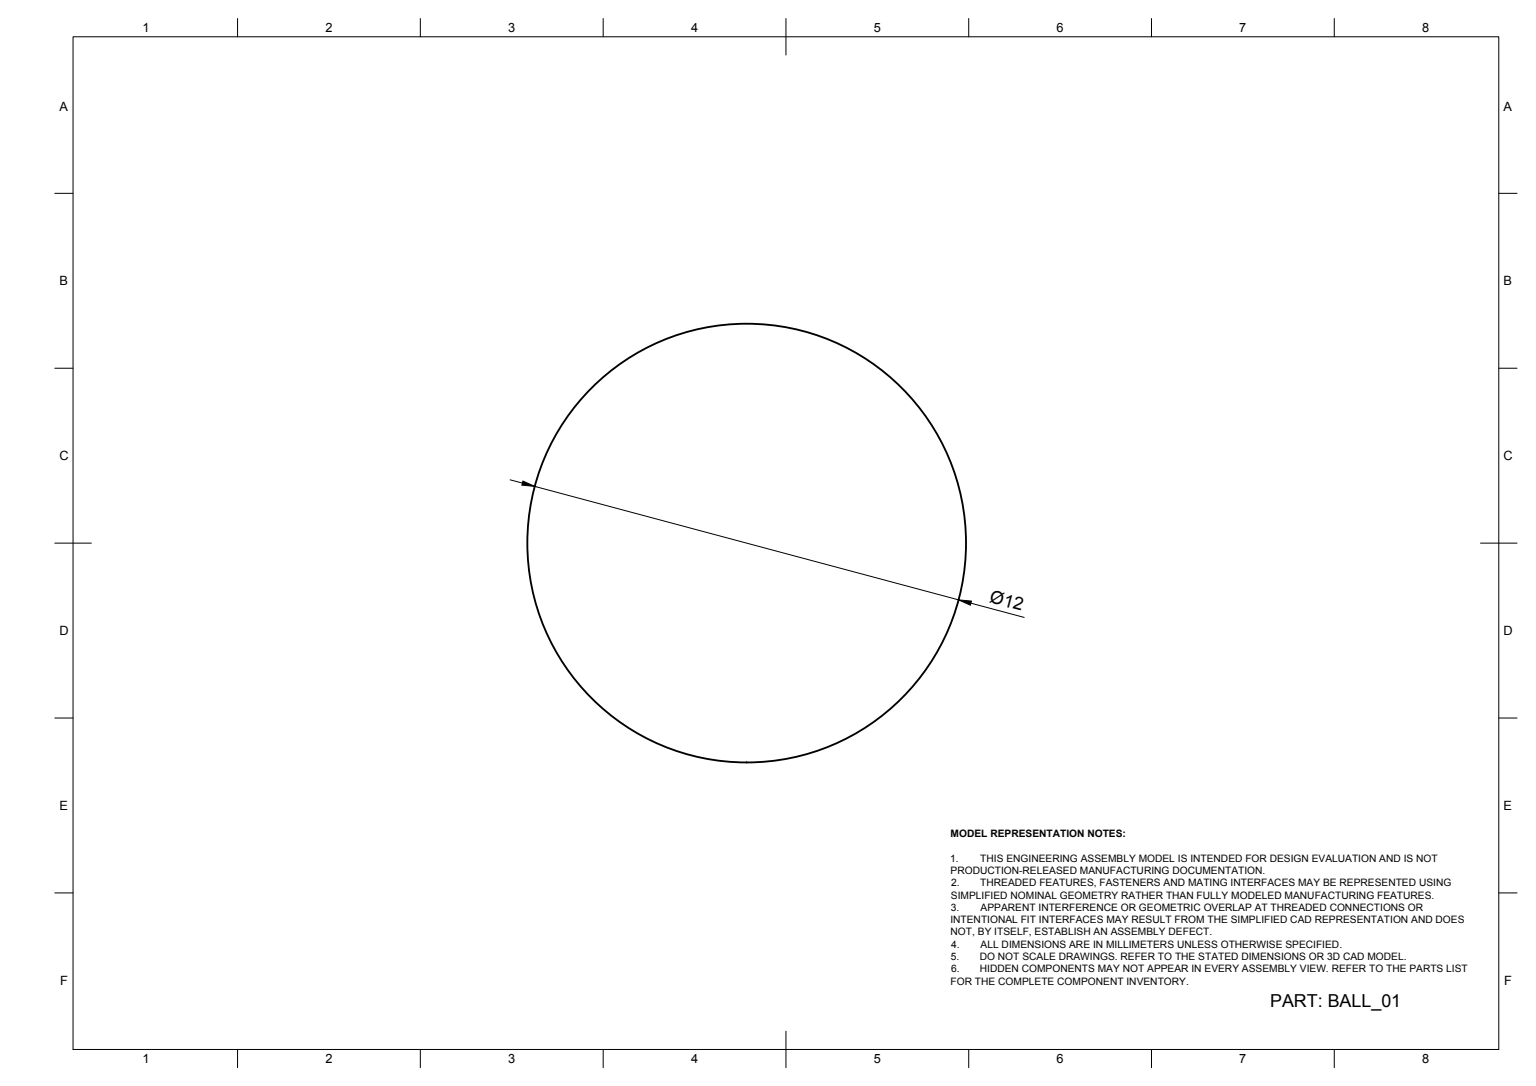
ISO-10303-21;
HEADER;
/* Generated by software containing ST-Developer
 * from STEP Tools, Inc. (www.steptools.com) 
 */

FILE_DESCRIPTION(
/* description */ (''),
/* implementation_level */ '2;1');

FILE_NAME(
/* name */ 'Ball_01.step',
/* time_stamp */ '2026-10-05T00:14:20-07:00',
/* author */ (''),
/* organization */ (''),
/* preprocessor_version */ 'ST-DEVELOPER v20.2',
/* originating_system */ 'Autodesk Translation Framework v15.15.0.0',
/* authorisation */ '');

FILE_SCHEMA (('AUTOMOTIVE_DESIGN { 1 0 10303 214 3 1 1 }'));
ENDSEC;

DATA;
#10=MECHANICAL_DESIGN_GEOMETRIC_PRESENTATION_REPRESENTATION('',(#3372),#75336);
#3352=SPHERICAL_SURFACE('',#32135,6.);
#3356=SHAPE_REPRESENTATION_RELATIONSHIP('SRR','None',#75369,#3364);
#3364=ADVANCED_BREP_SHAPE_REPRESENTATION('',(#3380),#75329);
#3372=STYLED_ITEM('',(#75418),#3380);
#3380=MANIFOLD_SOLID_BREP('Body1',#32022);
#3402=CIRCLE('',#32136,6.);
#5146=FACE_OUTER_BOUND('',#6874,.T.);
#6874=EDGE_LOOP('',(#19625,#19626));
#11108=VERTEX_POINT('',#46100);
#11109=VERTEX_POINT('',#46101);
#14507=EDGE_CURVE('',#11108,#11109,#3402,.T.);
#19625=ORIENTED_EDGE('',*,*,#14507,.T.);
#19626=ORIENTED_EDGE('',*,*,#14507,.F.);
#30306=ADVANCED_FACE('',(#5146),#3352,.T.);
#32022=CLOSED_SHELL('',(#30306));
#32134=AXIS2_PLACEMENT_3D('',#46098,#36399,#36400);
#32135=AXIS2_PLACEMENT_3D('',#46099,#36401,#36402);
#32136=AXIS2_PLACEMENT_3D('',#46102,#36403,#36404);
#36399=DIRECTION('axis',(0.,0.,1.));
#36400=DIRECTION('refdir',(1.,0.,0.));
#36401=DIRECTION('center_axis',(0.,0.,1.));
#36402=DIRECTION('ref_axis',(1.,0.,0.));
#36403=DIRECTION('center_axis',(1.22464679914735E-16,-1.,0.));
#36404=DIRECTION('ref_axis',(-1.,-1.22464679914735E-16,0.));
#46098=CARTESIAN_POINT('',(0.,0.,0.));
#46099=CARTESIAN_POINT('Origin',(30.,-9.99200722162641E-15,13.));
#46100=CARTESIAN_POINT('',(30.,-9.99200722162641E-15,19.));
#46101=CARTESIAN_POINT('',(30.,-9.99200722162641E-15,7.));
#46102=CARTESIAN_POINT('Origin',(30.,-9.99200722162641E-15,13.));
#75319=UNCERTAINTY_MEASURE_WITH_UNIT(LENGTH_MEASURE(0.01),#75337,
'DISTANCE_ACCURACY_VALUE',
'Maximum model space distance between geometric entities at asserted c
onnectivities');
#75326=UNCERTAINTY_MEASURE_WITH_UNIT(LENGTH_MEASURE(0.01),#75337,
'DISTANCE_ACCURACY_VALUE',
'Maximum model space distance between geometric entities at asserted c
onnectivities');
#75329=(
GEOMETRIC_REPRESENTATION_CONTEXT(3)
GLOBAL_UNCERTAINTY_ASSIGNED_CONTEXT((#75319))
GLOBAL_UNIT_ASSIGNED_CONTEXT((#75337,#75339,#75340))
REPRESENTATION_CONTEXT('','3D')
);
#75336=(
GEOMETRIC_REPRESENTATION_CONTEXT(3)
GLOBAL_UNCERTAINTY_ASSIGNED_CONTEXT((#75326))
GLOBAL_UNIT_ASSIGNED_CONTEXT((#75337,#75339,#75340))
REPRESENTATION_CONTEXT('','3D')
);
#75337=(
LENGTH_UNIT()
NAMED_UNIT(*)
SI_UNIT(.MILLI.,.METRE.)
);
#75339=(
NAMED_UNIT(*)
PLANE_ANGLE_UNIT()
SI_UNIT($,.RADIAN.)
);
#75340=(
NAMED_UNIT(*)
SI_UNIT($,.STERADIAN.)
SOLID_ANGLE_UNIT()
);
#75343=SHAPE_DEFINITION_REPRESENTATION(#75352,#75369);
#75352=PRODUCT_DEFINITION_SHAPE('',$,#75379);
#75369=SHAPE_REPRESENTATION('',(#32134),#75329);
#75376=PRODUCT_DEFINITION_CONTEXT('part definition',#75405,'design');
#75379=PRODUCT_DEFINITION('Ball_01','Ball_01',#75388,#75376);
#75388=PRODUCT_DEFINITION_FORMATION('',$,#75409);
#75405=APPLICATION_CONTEXT(
'Core Data for Automotive Mechanical Design Process');
#75406=PRODUCT_CONTEXT('part definition',#75405,'mechanical');
#75409=PRODUCT('Ball_01','Ball_01',$,(#75406));
#75418=PRESENTATION_STYLE_ASSIGNMENT((#75422));
#75422=SURFACE_STYLE_USAGE(.BOTH.,#75426);
#75426=SURFACE_SIDE_STYLE('',(#75430));
#75430=SURFACE_STYLE_FILL_AREA(#75434);
#75434=FILL_AREA_STYLE('Opaque(200,203,41)',(#75438));
#75438=FILL_AREA_STYLE_COLOUR('Opaque(200,203,41)',#75442);
#75442=COLOUR_RGB('Opaque(200,203,41)', 0.66274510, 0.83137255, 0.94901961);
ENDSEC;
END-ISO-10303-21;
